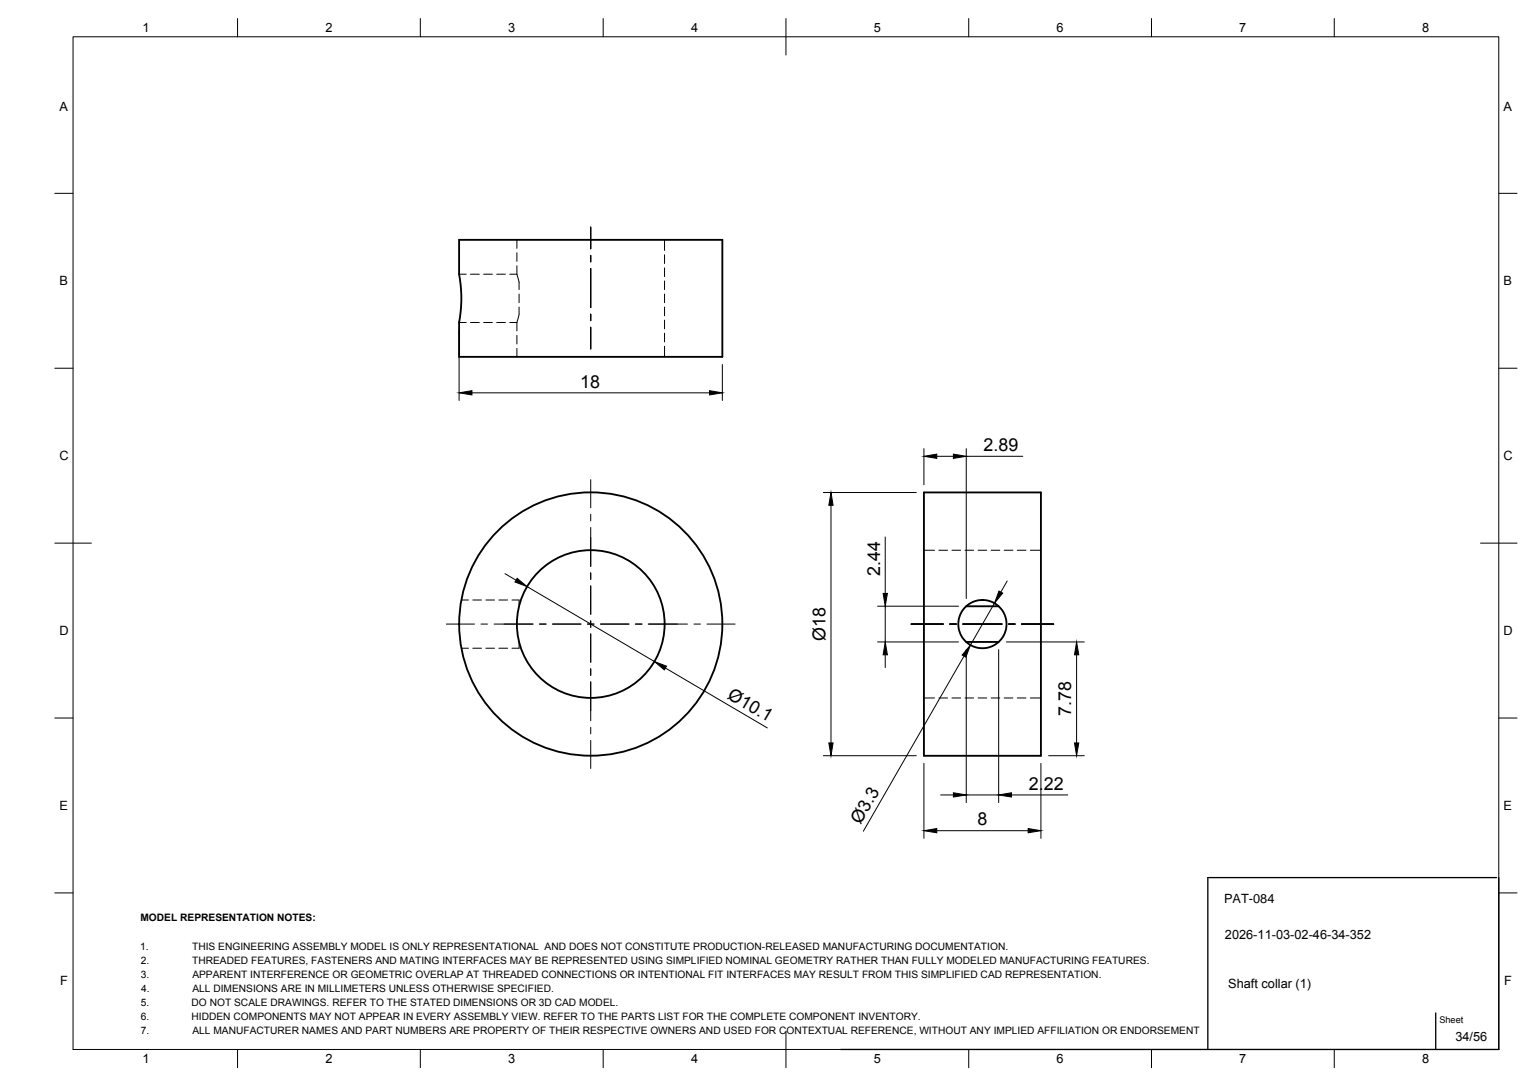
ISO-10303-21;
HEADER;
/* Generated by software containing ST-Developer
 * from STEP Tools, Inc. (www.steptools.com) 
 */

FILE_DESCRIPTION(
/* description */ ('Quick-return (Whitworth) mechanism'),
/* implementation_level */ '2;1');

FILE_NAME(
/* name */ 'Shaft collar (1).step',
/* time_stamp */ '2026-10-28T03:25:57-07:00',
/* author */ (''),
/* organization */ (''),
/* preprocessor_version */ 'ST-DEVELOPER v20.2',
/* originating_system */ 'Autodesk Translation Framework v15.17.0.0',
/* authorisation */ '');

FILE_SCHEMA (('AUTOMOTIVE_DESIGN { 1 0 10303 214 3 1 1 }'));
ENDSEC;

DATA;
#10=MECHANICAL_DESIGN_GEOMETRIC_PRESENTATION_REPRESENTATION('',(#522),#14878);
#397=B_SPLINE_CURVE_WITH_KNOTS('',3,(#13821,#13822,#13823,#13824,#13825,
#13826,#13827,#13828,#13829,#13830,#13831,#13832,#13833,#13834),
 .UNSPECIFIED.,.F.,.F.,(4,2,2,2,2,2,4),(0.618551524396293,0.626563103102765,
0.689203386094988,0.751843669087211,0.814483952079434,0.877124235071657,
0.88513581377813),.UNSPECIFIED.);
#398=B_SPLINE_CURVE_WITH_KNOTS('',3,(#13838,#13839,#13840,#13841,#13842,
#13843,#13844,#13845),.UNSPECIFIED.,.F.,.F.,(4,2,2,4),(0.250614556362404,
0.313254839354627,0.37589512234685,0.383906701053323),.UNSPECIFIED.);
#399=B_SPLINE_CURVE_WITH_KNOTS('',3,(#13849,#13850,#13851,#13852,#13853,
#13854,#13855,#13856,#13857,#13858,#13859,#13860,#13861,#13862,#13863,#13864,
#13865,#13866,#13867,#13868,#13869,#13870,#13871,#13872,#13873,#13874),
 .UNSPECIFIED.,.F.,.F.,(4,2,2,2,2,2,2,2,2,2,2,2,4),(0.,0.0623062782223143,
0.124612556444629,0.186916384615149,0.249220212785669,0.31152404095619,
0.37382786912671,0.436134147349024,0.498440425571339,0.560746703793653,
0.623052982015967,0.685356810186488,0.747660638357008),.UNSPECIFIED.);
#400=B_SPLINE_CURVE_WITH_KNOTS('',3,(#13875,#13876,#13877,#13878,#13879,
#13880,#13881,#13882,#13883,#13884),.UNSPECIFIED.,.F.,.F.,(4,2,2,2,4),(0.747660638357008,
0.809964466527528,0.872268294698049,0.934574572920363,0.996880851142677),
 .UNSPECIFIED.);
#401=B_SPLINE_CURVE_WITH_KNOTS('',3,(#13885,#13886,#13887,#13888,#13889,
#13890,#13891,#13892),.UNSPECIFIED.,.F.,.F.,(4,2,2,4),(0.117322411671485,
0.125333990377958,0.187974273370181,0.250614556362404),.UNSPECIFIED.);
#426=SHAPE_REPRESENTATION_RELATIONSHIP('SRR','None',#15097,#470);
#470=ADVANCED_BREP_SHAPE_REPRESENTATION('',(#573),#14854);
#522=STYLED_ITEM('',(#15406),#573);
#573=MANIFOLD_SOLID_BREP('Body1',#7877);
#733=FACE_BOUND('',#1949,.T.);
#734=FACE_BOUND('',#1951,.T.);
#735=FACE_BOUND('',#1953,.T.);
#736=FACE_BOUND('',#1955,.T.);
#924=PLANE('',#9017);
#925=PLANE('',#9021);
#926=PLANE('',#9028);
#927=PLANE('',#9029);
#1337=FACE_OUTER_BOUND('',#1945,.T.);
#1338=FACE_OUTER_BOUND('',#1946,.T.);
#1339=FACE_OUTER_BOUND('',#1947,.T.);
#1340=FACE_OUTER_BOUND('',#1948,.T.);
#1341=FACE_OUTER_BOUND('',#1950,.T.);
#1342=FACE_OUTER_BOUND('',#1952,.T.);
#1343=FACE_OUTER_BOUND('',#1954,.T.);
#1945=EDGE_LOOP('',(#6460,#6461));
#1946=EDGE_LOOP('',(#6462,#6463,#6464,#6465,#6466,#6467,#6468,#6469,#6470));
#1947=EDGE_LOOP('',(#6471,#6472));
#1948=EDGE_LOOP('',(#6473,#6474,#6475,#6476));
#1949=EDGE_LOOP('',(#6477,#6478,#6479,#6480,#6481));
#1950=EDGE_LOOP('',(#6482,#6483,#6484,#6485));
#1951=EDGE_LOOP('',(#6486,#6487));
#1952=EDGE_LOOP('',(#6488));
#1953=EDGE_LOOP('',(#6489));
#1954=EDGE_LOOP('',(#6490));
#1955=EDGE_LOOP('',(#6491));
#2430=LINE('',#13817,#2953);
#2431=LINE('',#13847,#2954);
#2432=LINE('',#13894,#2955);
#2433=LINE('',#13899,#2956);
#2434=LINE('',#13905,#2957);
#2953=VECTOR('',#10925,1.);
#2954=VECTOR('',#10932,0.165);
#2955=VECTOR('',#10935,1.);
#2956=VECTOR('',#10940,0.505);
#2957=VECTOR('',#10947,0.9);
#3524=CIRCLE('',#9018,0.165);
#3525=CIRCLE('',#9020,0.165);
#3526=CIRCLE('',#9023,0.505);
#3527=CIRCLE('',#9024,0.505);
#3528=CIRCLE('',#9026,0.9);
#3529=CIRCLE('',#9027,0.9);
#4040=VERTEX_POINT('',#13815);
#4041=VERTEX_POINT('',#13816);
#4042=VERTEX_POINT('',#13820);
#4043=VERTEX_POINT('',#13835);
#4044=VERTEX_POINT('',#13837);
#4045=VERTEX_POINT('',#13846);
#4046=VERTEX_POINT('',#13848);
#4047=VERTEX_POINT('',#13896);
#4048=VERTEX_POINT('',#13898);
#4049=VERTEX_POINT('',#13902);
#4050=VERTEX_POINT('',#13904);
#4887=EDGE_CURVE('',#4040,#4041,#2430,.T.);
#4888=EDGE_CURVE('',#4040,#4041,#3524,.T.);
#4889=EDGE_CURVE('',#4042,#4040,#397,.T.);
#4890=EDGE_CURVE('',#4043,#4042,#3525,.T.);
#4891=EDGE_CURVE('',#4044,#4043,#398,.T.);
#4892=EDGE_CURVE('',#4044,#4045,#2431,.T.);
#4893=EDGE_CURVE('',#4046,#4045,#399,.T.);
#4894=EDGE_CURVE('',#4045,#4046,#400,.T.);
#4895=EDGE_CURVE('',#4041,#4044,#401,.T.);
#4896=EDGE_CURVE('',#4043,#4042,#2432,.T.);
#4897=EDGE_CURVE('',#4047,#4047,#3526,.T.);
#4898=EDGE_CURVE('',#4047,#4048,#2433,.T.);
#4899=EDGE_CURVE('',#4048,#4048,#3527,.T.);
#4900=EDGE_CURVE('',#4049,#4049,#3528,.T.);
#4901=EDGE_CURVE('',#4049,#4050,#2434,.T.);
#4902=EDGE_CURVE('',#4050,#4050,#3529,.T.);
#6460=ORIENTED_EDGE('',*,*,#4887,.F.);
#6461=ORIENTED_EDGE('',*,*,#4888,.T.);
#6462=ORIENTED_EDGE('',*,*,#4889,.F.);
#6463=ORIENTED_EDGE('',*,*,#4890,.F.);
#6464=ORIENTED_EDGE('',*,*,#4891,.F.);
#6465=ORIENTED_EDGE('',*,*,#4892,.T.);
#6466=ORIENTED_EDGE('',*,*,#4893,.F.);
#6467=ORIENTED_EDGE('',*,*,#4894,.F.);
#6468=ORIENTED_EDGE('',*,*,#4892,.F.);
#6469=ORIENTED_EDGE('',*,*,#4895,.F.);
#6470=ORIENTED_EDGE('',*,*,#4888,.F.);
#6471=ORIENTED_EDGE('',*,*,#4896,.F.);
#6472=ORIENTED_EDGE('',*,*,#4890,.T.);
#6473=ORIENTED_EDGE('',*,*,#4897,.F.);
#6474=ORIENTED_EDGE('',*,*,#4898,.T.);
#6475=ORIENTED_EDGE('',*,*,#4899,.T.);
#6476=ORIENTED_EDGE('',*,*,#4898,.F.);
#6477=ORIENTED_EDGE('',*,*,#4895,.T.);
#6478=ORIENTED_EDGE('',*,*,#4891,.T.);
#6479=ORIENTED_EDGE('',*,*,#4896,.T.);
#6480=ORIENTED_EDGE('',*,*,#4889,.T.);
#6481=ORIENTED_EDGE('',*,*,#4887,.T.);
#6482=ORIENTED_EDGE('',*,*,#4900,.F.);
#6483=ORIENTED_EDGE('',*,*,#4901,.T.);
#6484=ORIENTED_EDGE('',*,*,#4902,.T.);
#6485=ORIENTED_EDGE('',*,*,#4901,.F.);
#6486=ORIENTED_EDGE('',*,*,#4893,.T.);
#6487=ORIENTED_EDGE('',*,*,#4894,.T.);
#6488=ORIENTED_EDGE('',*,*,#4900,.T.);
#6489=ORIENTED_EDGE('',*,*,#4897,.T.);
#6490=ORIENTED_EDGE('',*,*,#4902,.F.);
#6491=ORIENTED_EDGE('',*,*,#4899,.F.);
#7332=CYLINDRICAL_SURFACE('',#9019,0.165);
#7333=CYLINDRICAL_SURFACE('',#9022,0.505);
#7334=CYLINDRICAL_SURFACE('',#9025,0.9);
#7668=ADVANCED_FACE('',(#1337),#924,.T.);
#7669=ADVANCED_FACE('',(#1338),#7332,.F.);
#7670=ADVANCED_FACE('',(#1339),#925,.T.);
#7671=ADVANCED_FACE('',(#1340,#733),#7333,.F.);
#7672=ADVANCED_FACE('',(#1341,#734),#7334,.T.);
#7673=ADVANCED_FACE('',(#1342,#735),#926,.T.);
#7674=ADVANCED_FACE('',(#1343,#736),#927,.F.);
#7877=CLOSED_SHELL('',(#7668,#7669,#7670,#7671,#7672,#7673,#7674));
#9016=AXIS2_PLACEMENT_3D('',#13813,#10921,#10922);
#9017=AXIS2_PLACEMENT_3D('',#13814,#10923,#10924);
#9018=AXIS2_PLACEMENT_3D('',#13818,#10926,#10927);
#9019=AXIS2_PLACEMENT_3D('',#13819,#10928,#10929);
#9020=AXIS2_PLACEMENT_3D('',#13836,#10930,#10931);
#9021=AXIS2_PLACEMENT_3D('',#13893,#10933,#10934);
#9022=AXIS2_PLACEMENT_3D('',#13895,#10936,#10937);
#9023=AXIS2_PLACEMENT_3D('',#13897,#10938,#10939);
#9024=AXIS2_PLACEMENT_3D('',#13900,#10941,#10942);
#9025=AXIS2_PLACEMENT_3D('',#13901,#10943,#10944);
#9026=AXIS2_PLACEMENT_3D('',#13903,#10945,#10946);
#9027=AXIS2_PLACEMENT_3D('',#13906,#10948,#10949);
#9028=AXIS2_PLACEMENT_3D('',#13907,#10950,#10951);
#9029=AXIS2_PLACEMENT_3D('',#13908,#10952,#10953);
#10921=DIRECTION('axis',(0.,0.,1.));
#10922=DIRECTION('refdir',(1.,0.,0.));
#10923=DIRECTION('center_axis',(1.,0.,0.));
#10924=DIRECTION('ref_axis',(0.,0.,-1.));
#10925=DIRECTION('',(0.,0.,1.));
#10926=DIRECTION('center_axis',(1.,0.,0.));
#10927=DIRECTION('ref_axis',(0.,0.,-1.));
#10928=DIRECTION('center_axis',(1.,0.,0.));
#10929=DIRECTION('ref_axis',(0.,0.,-1.));
#10930=DIRECTION('center_axis',(1.,0.,0.));
#10931=DIRECTION('ref_axis',(0.,0.,-1.));
#10932=DIRECTION('',(1.,0.,0.));
#10933=DIRECTION('center_axis',(1.,0.,0.));
#10934=DIRECTION('ref_axis',(0.,0.,-1.));
#10935=DIRECTION('',(0.,0.,-1.));
#10936=DIRECTION('center_axis',(0.,0.,1.));
#10937=DIRECTION('ref_axis',(1.,0.,0.));
#10938=DIRECTION('center_axis',(0.,0.,-1.));
#10939=DIRECTION('ref_axis',(1.,0.,0.));
#10940=DIRECTION('',(0.,0.,-1.));
#10941=DIRECTION('center_axis',(0.,0.,-1.));
#10942=DIRECTION('ref_axis',(1.,0.,0.));
#10943=DIRECTION('center_axis',(0.,0.,1.));
#10944=DIRECTION('ref_axis',(1.,0.,0.));
#10945=DIRECTION('center_axis',(0.,0.,1.));
#10946=DIRECTION('ref_axis',(1.,0.,0.));
#10947=DIRECTION('',(0.,0.,-1.));
#10948=DIRECTION('center_axis',(0.,0.,1.));
#10949=DIRECTION('ref_axis',(1.,0.,0.));
#10950=DIRECTION('center_axis',(0.,0.,1.));
#10951=DIRECTION('ref_axis',(1.,0.,0.));
#10952=DIRECTION('center_axis',(0.,0.,1.));
#10953=DIRECTION('ref_axis',(1.,0.,0.));
#13813=CARTESIAN_POINT('',(0.,0.,0.));
#13814=CARTESIAN_POINT('Origin',(0.49,0.,1.4));
#13815=CARTESIAN_POINT('',(0.49,0.122167917228706,1.28909463493591));
#13816=CARTESIAN_POINT('',(0.49,0.122167917228706,1.51090536506409));
#13817=CARTESIAN_POINT('',(0.49,0.122167917228706,1.));
#13818=CARTESIAN_POINT('Origin',(0.49,0.,1.4));
#13819=CARTESIAN_POINT('Origin',(0.49,0.,1.4));
#13820=CARTESIAN_POINT('',(0.49,-0.122167917228706,1.28909463493591));
#13821=CARTESIAN_POINT('Ctrl Pts',(0.49,-0.122167917228706,1.28909463493591));
#13822=CARTESIAN_POINT('Ctrl Pts',(0.490448531679987,-0.120368913626296,
1.28711294069536));
#13823=CARTESIAN_POINT('Ctrl Pts',(0.490895245371685,-0.118534896565231,
1.28518965877367));
#13824=CARTESIAN_POINT('Ctrl Pts',(0.494795015531646,-0.102111993019358,
1.2687667552278));
#13825=CARTESIAN_POINT('Ctrl Pts',(0.498442514607594,-0.0836597150224318,
1.25609154388858));
#13826=CARTESIAN_POINT('Ctrl Pts',(0.50357781976106,-0.0430495960471595,
1.23920409039234));
#13827=CARTESIAN_POINT('Ctrl Pts',(0.505,-0.020880094330741,1.235));
#13828=CARTESIAN_POINT('Ctrl Pts',(0.505,0.020880094330741,1.235));
#13829=CARTESIAN_POINT('Ctrl Pts',(0.50357781976106,0.0430495960471595,
1.23920409039234));
#13830=CARTESIAN_POINT('Ctrl Pts',(0.498442514607594,0.0836597150224318,
1.25609154388858));
#13831=CARTESIAN_POINT('Ctrl Pts',(0.494795015531646,0.102111993019358,
1.2687667552278));
#13832=CARTESIAN_POINT('Ctrl Pts',(0.490895245371684,0.118534896565231,
1.28518965877367));
#13833=CARTESIAN_POINT('Ctrl Pts',(0.490448531679987,0.120368913626296,
1.28711294069536));
#13834=CARTESIAN_POINT('Ctrl Pts',(0.49,0.122167917228706,1.28909463493591));
#13835=CARTESIAN_POINT('',(0.49,-0.122167917228706,1.51090536506409));
#13836=CARTESIAN_POINT('Origin',(0.49,0.,1.4));
#13837=CARTESIAN_POINT('',(0.505,-1.70422299968729E-17,1.565));
#13838=CARTESIAN_POINT('Ctrl Pts',(0.505,-6.93889390390723E-18,1.565));
#13839=CARTESIAN_POINT('Ctrl Pts',(0.505,-0.020880094330741,1.565));
#13840=CARTESIAN_POINT('Ctrl Pts',(0.50357781976106,-0.0430495960471595,
1.56079590960766));
#13841=CARTESIAN_POINT('Ctrl Pts',(0.498442514607594,-0.0836597150224318,
1.54390845611142));
#13842=CARTESIAN_POINT('Ctrl Pts',(0.494795015531646,-0.102111993019358,
1.5312332447722));
#13843=CARTESIAN_POINT('Ctrl Pts',(0.490895245371684,-0.118534896565231,
1.51481034122633));
#13844=CARTESIAN_POINT('Ctrl Pts',(0.490448531679987,-0.120368913626296,
1.51288705930464));
#13845=CARTESIAN_POINT('Ctrl Pts',(0.49,-0.122167917228706,1.51090536506409));
#13846=CARTESIAN_POINT('',(0.9,-2.02066721859313E-17,1.565));
#13847=CARTESIAN_POINT('',(0.49,-2.02066721859313E-17,1.565));
#13848=CARTESIAN_POINT('',(0.884745726183518,0.165,1.4));
#13849=CARTESIAN_POINT('Ctrl Pts',(0.884745726183518,0.165,1.4));
#13850=CARTESIAN_POINT('Ctrl Pts',(0.884745726183518,0.165,1.37923124059256));
#13851=CARTESIAN_POINT('Ctrl Pts',(0.885552759505264,0.160839719007584,
1.35711110492666));
#13852=CARTESIAN_POINT('Ctrl Pts',(0.888448648150043,0.143986470216691,
1.31647293736623));
#13853=CARTESIAN_POINT('Ctrl Pts',(0.890493604851638,0.131295993814186,
1.29795075602263));
#13854=CARTESIAN_POINT('Ctrl Pts',(0.89431723432394,0.102049819008125,1.26870458121656));
#13855=CARTESIAN_POINT('Ctrl Pts',(0.896347088899543,0.0835273920906824,
1.25601365401642));
#13856=CARTESIAN_POINT('Ctrl Pts',(0.899208271860583,0.0428883760934127,
1.23916007816136));
#13857=CARTESIAN_POINT('Ctrl Pts',(0.9,0.0207679427235068,1.235));
#13858=CARTESIAN_POINT('Ctrl Pts',(0.9,-0.0207679427235068,1.235));
#13859=CARTESIAN_POINT('Ctrl Pts',(0.899208271860583,-0.0428883760934127,
1.23916007816136));
#13860=CARTESIAN_POINT('Ctrl Pts',(0.896347088899543,-0.0835273920906823,
1.25601365401642));
#13861=CARTESIAN_POINT('Ctrl Pts',(0.89431723432394,-0.102049819008125,
1.26870458121656));
#13862=CARTESIAN_POINT('Ctrl Pts',(0.890493604851638,-0.131295993814186,
1.29795075602263));
#13863=CARTESIAN_POINT('Ctrl Pts',(0.888448648150043,-0.143986470216691,
1.31647293736623));
#13864=CARTESIAN_POINT('Ctrl Pts',(0.885552759505264,-0.160839719007584,
1.35711110492666));
#13865=CARTESIAN_POINT('Ctrl Pts',(0.884745726183518,-0.165,1.37923124059256));
#13866=CARTESIAN_POINT('Ctrl Pts',(0.884745726183518,-0.165,1.42076875940744));
#13867=CARTESIAN_POINT('Ctrl Pts',(0.885552759505264,-0.160839719007584,
1.44288889507334));
#13868=CARTESIAN_POINT('Ctrl Pts',(0.888448648150043,-0.14398647021669,
1.48352706263377));
#13869=CARTESIAN_POINT('Ctrl Pts',(0.890493604851638,-0.131295993814186,
1.50204924397737));
#13870=CARTESIAN_POINT('Ctrl Pts',(0.89431723432394,-0.102049819008125,
1.53129541878344));
#13871=CARTESIAN_POINT('Ctrl Pts',(0.896347088899543,-0.0835273920906824,
1.54398634598358));
#13872=CARTESIAN_POINT('Ctrl Pts',(0.899208271860583,-0.0428883760934128,
1.56083992183864));
#13873=CARTESIAN_POINT('Ctrl Pts',(0.9,-0.0207679427235068,1.565));
#13874=CARTESIAN_POINT('Ctrl Pts',(0.9,-6.93889390390723E-18,1.565));
#13875=CARTESIAN_POINT('Ctrl Pts',(0.9,-3.46944695195361E-17,1.565));
#13876=CARTESIAN_POINT('Ctrl Pts',(0.9,0.0207679427235068,1.565));
#13877=CARTESIAN_POINT('Ctrl Pts',(0.899208271860583,0.0428883760934127,
1.56083992183864));
#13878=CARTESIAN_POINT('Ctrl Pts',(0.896347088899543,0.0835273920906824,
1.54398634598358));
#13879=CARTESIAN_POINT('Ctrl Pts',(0.89431723432394,0.102049819008125,1.53129541878344));
#13880=CARTESIAN_POINT('Ctrl Pts',(0.890493604851638,0.131295993814186,
1.50204924397737));
#13881=CARTESIAN_POINT('Ctrl Pts',(0.888448648150043,0.143986470216691,
1.48352706263377));
#13882=CARTESIAN_POINT('Ctrl Pts',(0.885552759505264,0.160839719007584,
1.44288889507334));
#13883=CARTESIAN_POINT('Ctrl Pts',(0.884745726183518,0.165,1.42076875940744));
#13884=CARTESIAN_POINT('Ctrl Pts',(0.884745726183518,0.165,1.4));
#13885=CARTESIAN_POINT('Ctrl Pts',(0.49,0.122167917228706,1.51090536506409));
#13886=CARTESIAN_POINT('Ctrl Pts',(0.490448531679987,0.120368913626296,
1.51288705930464));
#13887=CARTESIAN_POINT('Ctrl Pts',(0.490895245371685,0.118534896565231,
1.51481034122633));
#13888=CARTESIAN_POINT('Ctrl Pts',(0.494795015531646,0.102111993019358,
1.5312332447722));
#13889=CARTESIAN_POINT('Ctrl Pts',(0.498442514607594,0.0836597150224318,
1.54390845611142));
#13890=CARTESIAN_POINT('Ctrl Pts',(0.50357781976106,0.0430495960471594,
1.56079590960766));
#13891=CARTESIAN_POINT('Ctrl Pts',(0.505,0.020880094330741,1.565));
#13892=CARTESIAN_POINT('Ctrl Pts',(0.505,0.,1.565));
#13893=CARTESIAN_POINT('Origin',(0.49,0.,1.4));
#13894=CARTESIAN_POINT('',(0.49,-0.122167917228706,1.));
#13895=CARTESIAN_POINT('Origin',(0.,0.,1.));
#13896=CARTESIAN_POINT('',(-0.505,-6.18446633569413E-17,1.8));
#13897=CARTESIAN_POINT('Origin',(0.,0.,1.8));
#13898=CARTESIAN_POINT('',(-0.505,-6.18446633569413E-17,1.));
#13899=CARTESIAN_POINT('',(-0.505,-6.18446633569413E-17,1.));
#13900=CARTESIAN_POINT('Origin',(0.,0.,1.));
#13901=CARTESIAN_POINT('Origin',(0.,0.,1.));
#13902=CARTESIAN_POINT('',(-0.9,-1.10218211923262E-16,1.8));
#13903=CARTESIAN_POINT('Origin',(0.,0.,1.8));
#13904=CARTESIAN_POINT('',(-0.9,-1.10218211923262E-16,1.));
#13905=CARTESIAN_POINT('',(-0.9,-1.10218211923262E-16,1.));
#13906=CARTESIAN_POINT('Origin',(0.,0.,1.));
#13907=CARTESIAN_POINT('Origin',(0.,0.,1.8));
#13908=CARTESIAN_POINT('Origin',(0.,0.,1.));
#14800=UNCERTAINTY_MEASURE_WITH_UNIT(LENGTH_MEASURE(0.001),#14879,
'DISTANCE_ACCURACY_VALUE',
'Maximum model space distance between geometric entities at asserted c
onnectivities');
#14824=UNCERTAINTY_MEASURE_WITH_UNIT(LENGTH_MEASURE(0.001),#14879,
'DISTANCE_ACCURACY_VALUE',
'Maximum model space distance between geometric entities at asserted c
onnectivities');
#14854=(
GEOMETRIC_REPRESENTATION_CONTEXT(3)
GLOBAL_UNCERTAINTY_ASSIGNED_CONTEXT((#14800))
GLOBAL_UNIT_ASSIGNED_CONTEXT((#14879,#14881,#14882))
REPRESENTATION_CONTEXT('','3D')
);
#14878=(
GEOMETRIC_REPRESENTATION_CONTEXT(3)
GLOBAL_UNCERTAINTY_ASSIGNED_CONTEXT((#14824))
GLOBAL_UNIT_ASSIGNED_CONTEXT((#14879,#14881,#14882))
REPRESENTATION_CONTEXT('','3D')
);
#14879=(
LENGTH_UNIT()
NAMED_UNIT(*)
SI_UNIT(.CENTI.,.METRE.)
);
#14881=(
NAMED_UNIT(*)
PLANE_ANGLE_UNIT()
SI_UNIT($,.RADIAN.)
);
#14882=(
NAMED_UNIT(*)
SI_UNIT($,.STERADIAN.)
SOLID_ANGLE_UNIT()
);
#14912=SHAPE_DEFINITION_REPRESENTATION(#14970,#15097);
#14970=PRODUCT_DEFINITION_SHAPE('',$,#15151);
#15097=SHAPE_REPRESENTATION('',(#9016),#14854);
#15121=PRODUCT_DEFINITION_CONTEXT('part definition',#15282,'design');
#15151=PRODUCT_DEFINITION('Shaft collar (1)','Shaft collar (1)',#15204,#15121);
#15204=PRODUCT_DEFINITION_FORMATION('',$,#15313);
#15282=APPLICATION_CONTEXT(
'Core Data for Automotive Mechanical Design Process');
#15283=PRODUCT_CONTEXT('part definition',#15282,'mechanical');
#15313=PRODUCT('Shaft collar (1)','Shaft collar (1)','Shaft collar (1)',(#15283));
#15400=COLOUR_RGB('Grey',0.48,0.52,0.57);
#15401=FILL_AREA_STYLE_COLOUR('',#15400);
#15402=FILL_AREA_STYLE('',(#15401));
#15403=SURFACE_STYLE_FILL_AREA(#15402);
#15404=SURFACE_SIDE_STYLE('',(#15403));
#15405=SURFACE_STYLE_USAGE(.BOTH.,#15404);
#15406=PRESENTATION_STYLE_ASSIGNMENT((#15405));
ENDSEC;
END-ISO-10303-21;
